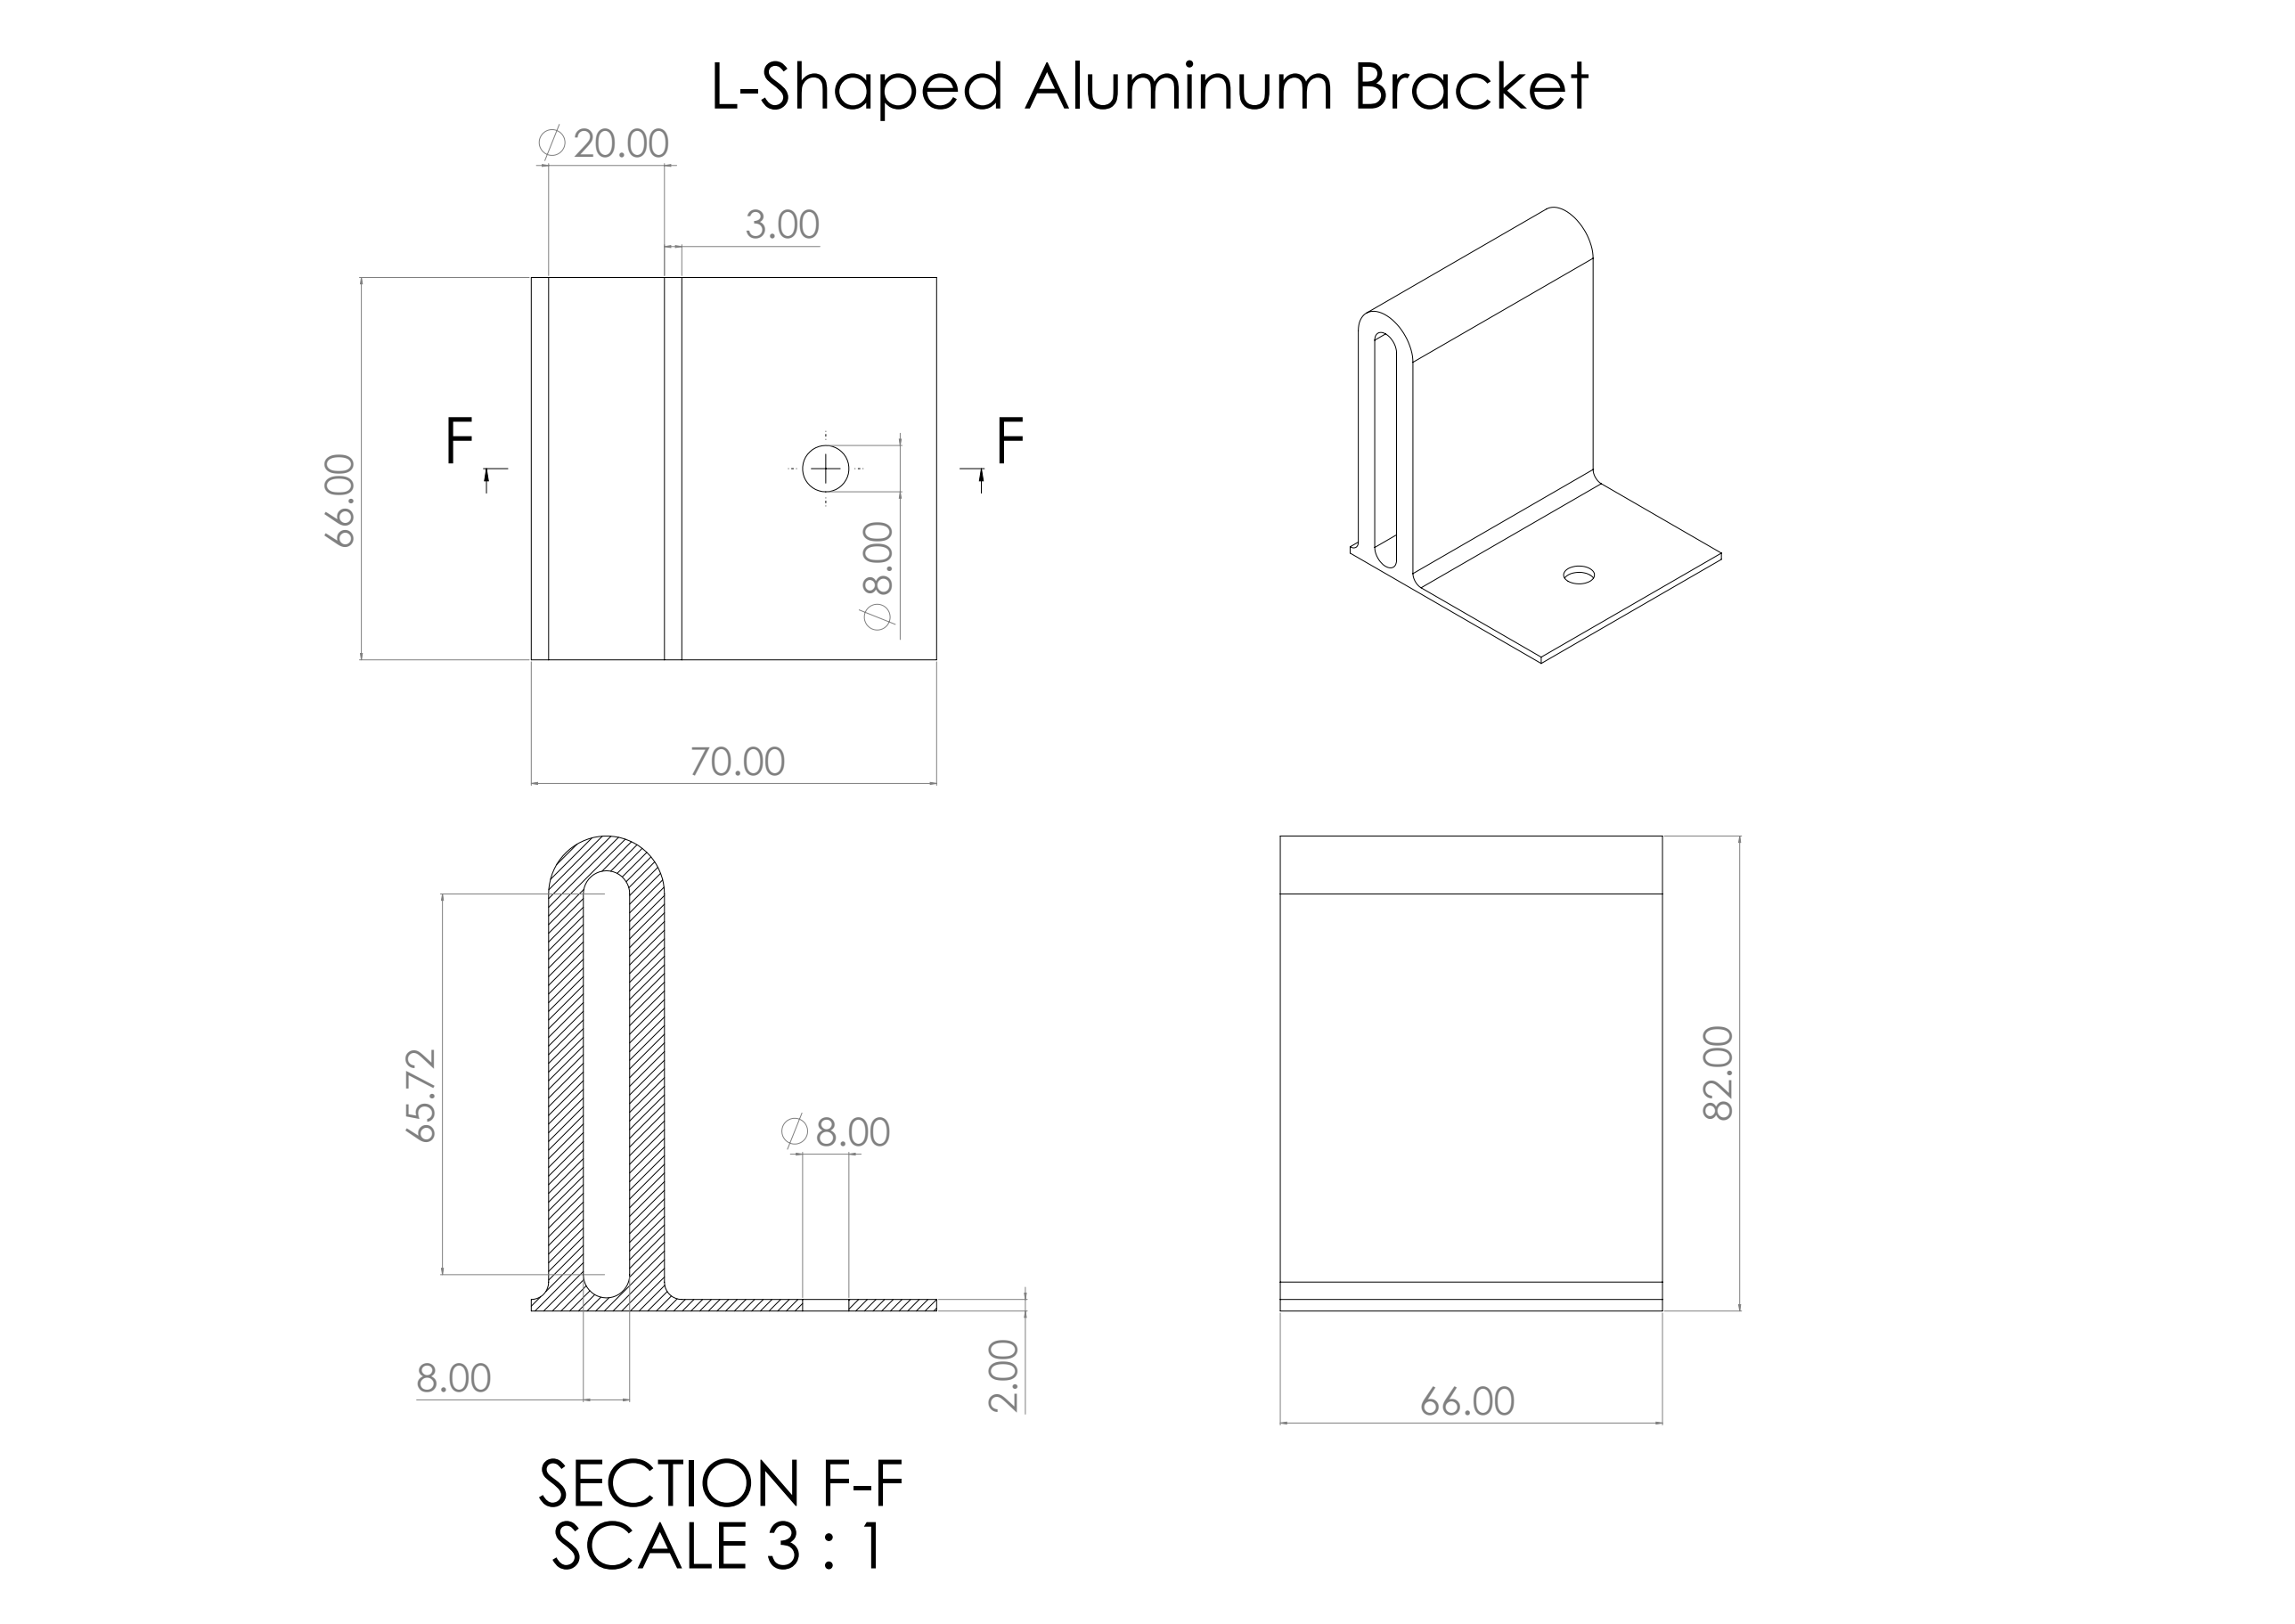
ISO-10303-21;
HEADER;
FILE_DESCRIPTION (('STEP AP214'),
    '1' );
FILE_NAME ('L-Shaped Aluminum Bracket.step',
    '2026-10-24T21:31:31',
    ( '' ),
    ( '' ),
    'SwSTEP 2.0',
    'SolidWorks 2025',
    '' );
FILE_SCHEMA (( 'AUTOMOTIVE_DESIGN' ));
ENDSEC;

DATA;
#12=EDGE_CURVE ( 'NONE', #11983, #7767, #13962, .T. ) ;
#46=PLANE ( 'NONE',  #3626 ) ;
#58=VECTOR ( 'NONE', #2580, 1000.000000000000000 ) ;
#63=DIRECTION ( 'NONE',  ( 0.000000000000000000, 1.734723475976817547E-15, -1.000000000000000000 ) ) ;
#73=EDGE_CURVE ( 'NONE', #927, #9462, #501, .T. ) ;
#97=AXIS2_PLACEMENT_3D ( 'NONE', #6521, #12302, #1688 ) ;
#99=CARTESIAN_POINT ( 'NONE',  ( 40.00000000000001421, -72.24929059928631148, -32.99999999999982947 ) ) ;
#111=FACE_OUTER_BOUND ( 'NONE', #10692, .T. ) ;
#122=EDGE_CURVE ( 'NONE', #12222, #13012, #6096, .T. ) ;
#154=DIRECTION ( 'NONE',  ( -0.000000000000000000, 1.000000000000000000, -0.000000000000000000 ) ) ;
#166=VERTEX_POINT ( 'NONE', #3346 ) ;
#182=FACE_OUTER_BOUND ( 'NONE', #8671, .T. ) ;
#200=CLOSED_SHELL ( 'NONE', ( #3830, #2727, #245, #8105, #11848, #11362, #3505, #1082, #828, #2082, #3069, #6755, #8169, #6132, #6771, #8839, #9223 ) ) ;
#204=ORIENTED_EDGE ( 'NONE', *, *, #247, .F. ) ;
#208=DIRECTION ( 'NONE',  ( -2.102695122396130409E-16, 0.000000000000000000, -1.000000000000000000 ) ) ;
#223=DIRECTION ( 'NONE',  ( 9.912705577010325549E-17, -1.734723475976817547E-15, 1.000000000000000000 ) ) ;
#245=ADVANCED_FACE ( 'NONE', ( #4003, #4739 ), #46, .F. ) ;
#247=EDGE_CURVE ( 'NONE', #8031, #13187, #10874, .T. ) ;
#263=CARTESIAN_POINT ( 'NONE',  ( -6.999999999999985789, -2.249290599286299930, -115.4621125123531442 ) ) ;
#286=VECTOR ( 'NONE', #5569, 1000.000000000000000 ) ;
#337=CARTESIAN_POINT ( 'NONE',  ( -26.99999999999998224, -72.24929059928645358, -33.00000000000000000 ) ) ;
#354=CARTESIAN_POINT ( 'NONE',  ( -29.99999999999998579, -72.24929059928631148, 33.00000000000000000 ) ) ;
#366=DIRECTION ( 'NONE',  ( 0.000000000000000000, 1.000000000000000000, 2.081668171172168119E-15 ) ) ;
#400=CARTESIAN_POINT ( 'NONE',  ( 80.00000000000001421, -72.24929059928631148, -32.99999999999999289 ) ) ;
#433=AXIS2_PLACEMENT_3D ( 'NONE', #3532, #9698, #7289 ) ;
#441=ORIENTED_EDGE ( 'NONE', *, *, #2442, .F. ) ;
#467=DIRECTION ( 'NONE',  ( 0.000000000000000000, 1.000000000000000000, 1.734723475976817547E-15 ) ) ;
#501=LINE ( 'NONE', #5201, #10269 ) ;
#520=VECTOR ( 'NONE', #3953, 1000.000000000000000 ) ;
#527=ORIENTED_EDGE ( 'NONE', *, *, #4321, .T. ) ;
#533=STYLED_ITEM('',(#15244),#4356);
#555=CARTESIAN_POINT ( 'NONE',  ( 20.86173033120691045, -74.24929059928636832, -3.999999999999999112 ) ) ;
#559=( NAMED_UNIT ( * ) SI_UNIT ( $, .STERADIAN. ) SOLID_ANGLE_UNIT ( ) );
#561=EDGE_CURVE ( 'NONE', #3921, #10500, #8809, .T. ) ;
#596=DIRECTION ( 'NONE',  ( -9.912705577010325549E-17, 1.734723475976817547E-15, -1.000000000000000000 ) ) ;
#602=LINE ( 'NONE', #8916, #9558 ) ;
#709=PLANE ( 'NONE',  #9602 ) ;
#714=DIRECTION ( 'NONE',  ( 0.000000000000000000, 0.000000000000000000, 1.000000000000000000 ) ) ;
#774=CARTESIAN_POINT ( 'NONE',  ( -29.99999999999998579, -74.24929059928642516, 32.99999999999999289 ) ) ;
#780=EDGE_CURVE ( 'NONE', #1026, #927, #5885, .T. ) ;
#802=FACE_BOUND ( 'NONE', #1169, .T. ) ;
#817=ORIENTED_EDGE ( 'NONE', *, *, #5665, .F. ) ;
#828=ADVANCED_FACE ( 'NONE', ( #11712 ), #13872, .T. ) ;
#927=VERTEX_POINT ( 'NONE', #5454 ) ;
#958=DIRECTION ( 'NONE',  ( -9.912705577010325549E-17, 1.734723475976817547E-15, -1.000000000000000000 ) ) ;
#965=VERTEX_POINT ( 'NONE', #11361 ) ;
#1000=EDGE_LOOP ( 'NONE', ( #9467, #6469, #14232, #3569 ) ) ;
#1019=VECTOR ( 'NONE', #8713, 1000.000000000000000 ) ;
#1026=VERTEX_POINT ( 'NONE', #8983 ) ;
#1027=VECTOR ( 'NONE', #1162, 1000.000000000000000 ) ;
#1061=CARTESIAN_POINT ( 'NONE',  ( 20.86173033120691045, -72.24929059928631148, -3.999999999999999112 ) ) ;
#1082=ADVANCED_FACE ( 'NONE', ( #8143 ), #6990, .T. ) ;
#1084=EDGE_CURVE ( 'NONE', #4458, #166, #5687, .T. ) ;
#1100=ORIENTED_EDGE ( 'NONE', *, *, #561, .F. ) ;
#1141=DIRECTION ( 'NONE',  ( -0.000000000000000000, -1.000000000000000000, -1.734723475976817547E-15 ) ) ;
#1161=ORIENTED_EDGE ( 'NONE', *, *, #780, .F. ) ;
#1162=DIRECTION ( 'NONE',  ( 1.051347561198064835E-16, 0.000000000000000000, 1.000000000000000000 ) ) ;
#1169=EDGE_LOOP ( 'NONE', ( #1100, #441 ) ) ;
#1181=CARTESIAN_POINT ( 'NONE',  ( 20.86173033120691045, -87.24929059928631148, 0.000000000000000000 ) ) ;
#1202=DIRECTION ( 'NONE',  ( 1.000000000000000000, 3.647594591642515023E-31, -2.102695122396130409E-16 ) ) ;
#1210=ORIENTED_EDGE ( 'NONE', *, *, #3031, .T. ) ;
#1211=CARTESIAN_POINT ( 'NONE',  ( -6.999999999999987566, -2.249290599286300818, -115.4621125123531442 ) ) ;
#1212=CARTESIAN_POINT ( 'NONE',  ( -16.99999999999998579, -67.96969602390581144, -115.4621125123531442 ) ) ;
#1224=CARTESIAN_POINT ( 'NONE',  ( -30.00000000000000000, 23.95881716715930665, -32.99999999999982236 ) ) ;
#1302=ORIENTED_EDGE ( 'NONE', *, *, #11228, .F. ) ;
#1315=ORIENTED_EDGE ( 'NONE', *, *, #6502, .T. ) ;
#1345=CARTESIAN_POINT ( 'NONE',  ( -12.99999999999998757, -2.249290599286444703, -32.99999999999987921 ) ) ;
#1422=AXIS2_PLACEMENT_3D ( 'NONE', #9838, #14588, #4037 ) ;
#1431=LINE ( 'NONE', #1654, #13791 ) ;
#1493=( LENGTH_UNIT ( ) NAMED_UNIT ( * ) SI_UNIT ( .MILLI., .METRE. ) );
#1522=CIRCLE ( 'NONE', #14296, 10.00000000000000178 ) ;
#1576=CARTESIAN_POINT ( 'NONE',  ( -6.999999999999978684, -69.24929059928631148, -32.99999999999999289 ) ) ;
#1624=CARTESIAN_POINT ( 'NONE',  ( -20.99999999999998579, -2.249290599286445591, -32.99999999999987921 ) ) ;
#1654=CARTESIAN_POINT ( 'NONE',  ( 40.00000000000002132, 23.95881716715919652, 33.00000000000017053 ) ) ;
#1658=ORIENTED_EDGE ( 'NONE', *, *, #11767, .F. ) ;
#1688=DIRECTION ( 'NONE',  ( 0.000000000000000000, 1.000000000000000000, 1.734723475976807094E-15 ) ) ;
#1716=DIRECTION ( 'NONE',  ( 0.000000000000000000, -1.000000000000000000, -2.312964634635740689E-15 ) ) ;
#1725=CIRCLE ( 'NONE', #14018, 3.000000000000002665 ) ;
#1728=ORIENTED_EDGE ( 'NONE', *, *, #247, .T. ) ;
#1747=CARTESIAN_POINT ( 'NONE',  ( 40.00000000000001421, 23.95881716715930665, -32.99999999999982947 ) ) ;
#1821=DIRECTION ( 'NONE',  ( 0.000000000000000000, 0.000000000000000000, 1.000000000000000000 ) ) ;
#1870=DIRECTION ( 'NONE',  ( -1.051347561198064835E-16, 1.682156097916903736E-15, -1.000000000000000000 ) ) ;
#2046=ORIENTED_EDGE ( 'NONE', *, *, #8831, .F. ) ;
#2067=ORIENTED_EDGE ( 'NONE', *, *, #10207, .F. ) ;
#2082=ADVANCED_FACE ( 'NONE', ( #14130 ), #2348, .T. ) ;
#2098=VECTOR ( 'NONE', #13951, 1000.000000000000000 ) ;
#2168=DIRECTION ( 'NONE',  ( 0.000000000000000000, 0.000000000000000000, 1.000000000000000000 ) ) ;
#2172=CARTESIAN_POINT ( 'NONE',  ( 20.86173033120691045, -72.24929059928631148, 0.000000000000000000 ) ) ;
#2185=ORIENTED_EDGE ( 'NONE', *, *, #780, .T. ) ;
#2190=LINE ( 'NONE', #13651, #9161 ) ;
#2193=AXIS2_PLACEMENT_3D ( 'NONE', #9260, #3255, #9025 ) ;
#2234=CARTESIAN_POINT ( 'NONE',  ( -20.99999999999998579, -67.96969602390581144, -32.99999999999998579 ) ) ;
#2255=CARTESIAN_POINT ( 'NONE',  ( 20.86173033120691045, -74.24929059928636832, 3.999999999999999112 ) ) ;
#2280=VERTEX_POINT ( 'NONE', #2234 ) ;
#2303=EDGE_LOOP ( 'NONE', ( #5933, #14533, #2769, #11027 ) ) ;
#2348=PLANE ( 'NONE',  #6120 ) ;
#2403=CARTESIAN_POINT ( 'NONE',  ( -6.999999999999978684, -69.24929059928631148, 33.00000000000000711 ) ) ;
#2420=ORIENTED_EDGE ( 'NONE', *, *, #3031, .F. ) ;
#2442=EDGE_CURVE ( 'NONE', #10500, #3921, #13064, .T. ) ;
#2445=CARTESIAN_POINT ( 'NONE',  ( -20.99999999999998579, -67.96969602390581144, -115.4621125123531442 ) ) ;
#2451=ORIENTED_EDGE ( 'NONE', *, *, #6579, .T. ) ;
#2475=ORIENTED_EDGE ( 'NONE', *, *, #7070, .F. ) ;
#2580=DIRECTION ( 'NONE',  ( 0.000000000000000000, -1.000000000000000000, -1.734723475976817547E-15 ) ) ;
#2610=ORIENTED_EDGE ( 'NONE', *, *, #13697, .F. ) ;
#2654=LINE ( 'NONE', #13195, #3969 ) ;
#2657=AXIS2_PLACEMENT_3D ( 'NONE', #13816, #958, #13740 ) ;
#2693=CARTESIAN_POINT ( 'NONE',  ( 20.86173033120691045, -74.24929059928636832, 0.000000000000000000 ) ) ;
#2727=ADVANCED_FACE ( 'NONE', ( #802, #13895 ), #5587, .T. ) ;
#2742=AXIS2_PLACEMENT_3D ( 'NONE', #12942, #12000, #10937 ) ;
#2744=DIRECTION ( 'NONE',  ( 0.000000000000000000, 1.734723475976817547E-15, -1.000000000000000000 ) ) ;
#2763=DIRECTION ( 'NONE',  ( 1.051347561198064835E-16, 0.000000000000000000, 1.000000000000000000 ) ) ;
#2769=ORIENTED_EDGE ( 'NONE', *, *, #10207, .T. ) ;
#2863=( LENGTH_UNIT ( ) NAMED_UNIT ( * ) SI_UNIT ( .MILLI., .METRE. ) );
#2902=DIRECTION ( 'NONE',  ( 0.000000000000000000, 1.734723475976817547E-15, -1.000000000000000000 ) ) ;
#2958=EDGE_LOOP ( 'NONE', ( #7879, #14398, #10143, #14155, #8547, #1210, #8196, #2978, #2185 ) ) ;
#2978=ORIENTED_EDGE ( 'NONE', *, *, #11176, .T. ) ;
#2982=CYLINDRICAL_SURFACE ( 'NONE', #15001, 2.999999999999999112 ) ;
#2999=CARTESIAN_POINT ( 'NONE',  ( -6.999999999999987566, -2.249290599286157821, 33.00000000000012790 ) ) ;
#3027=VERTEX_POINT ( 'NONE', #1576 ) ;
#3031=EDGE_CURVE ( 'NONE', #3027, #4458, #13994, .T. ) ;
#3040=VERTEX_POINT ( 'NONE', #12340 ) ;
#3047=DIRECTION ( 'NONE',  ( 2.102695122396130163E-16, -1.682156097916904130E-15, 1.000000000000000000 ) ) ;
#3069=ADVANCED_FACE ( 'NONE', ( #9190 ), #15111, .F. ) ;
#3142=ORIENTED_EDGE ( 'NONE', *, *, #13697, .T. ) ;
#3198=ORIENTED_EDGE ( 'NONE', *, *, #14960, .T. ) ;
#3227=AXIS2_PLACEMENT_3D ( 'NONE', #4760, #9745, #4598 ) ;
#3255=DIRECTION ( 'NONE',  ( -1.000000000000000000, 0.000000000000000000, 0.000000000000000000 ) ) ;
#3261=PRODUCT_DEFINITION ( 'UNKNOWN', '', #14928, #10440 ) ;
#3291=ORIENTED_EDGE ( 'NONE', *, *, #73, .T. ) ;
#3327=DIRECTION ( 'NONE',  ( 0.000000000000000000, 0.000000000000000000, 1.000000000000000000 ) ) ;
#3346=CARTESIAN_POINT ( 'NONE',  ( 40.00000000000001421, -72.24929059928631148, -32.99999999999999289 ) ) ;
#3408=CARTESIAN_POINT ( 'NONE',  ( -16.99999999999998579, -2.249290599286305703, -115.4621125123531442 ) ) ;
#3427=DIRECTION ( 'NONE',  ( 0.000000000000000000, -1.000000000000000000, -1.734723475976807094E-15 ) ) ;
#3484=DIRECTION ( 'NONE',  ( -1.000000000000000000, 0.000000000000000000, 9.912705577010325549E-17 ) ) ;
#3505=ADVANCED_FACE ( 'NONE', ( #9807, #182 ), #14348, .F. ) ;
#3532=CARTESIAN_POINT ( 'NONE',  ( -3.999999999999976019, -69.24929059928631148, -32.99999999999999289 ) ) ;
#3552=ORIENTED_EDGE ( 'NONE', *, *, #7518, .T. ) ;
#3564=CYLINDRICAL_SURFACE ( 'NONE', #7608, 3.999999999999999112 ) ;
#3569=ORIENTED_EDGE ( 'NONE', *, *, #14929, .T. ) ;
#3603=CARTESIAN_POINT ( 'NONE',  ( -29.99999999999998224, -69.24929059928631148, -32.99999999999998579 ) ) ;
#3626=AXIS2_PLACEMENT_3D ( 'NONE', #8701, #14129, #13391 ) ;
#3717=ORIENTED_EDGE ( 'NONE', *, *, #7737, .F. ) ;
#3801=LINE ( 'NONE', #8505, #1019 ) ;
#3830=ADVANCED_FACE ( 'NONE', ( #13277 ), #12119, .F. ) ;
#3845=VECTOR ( 'NONE', #14312, 1000.000000000000000 ) ;
#3854=EDGE_CURVE ( 'NONE', #2280, #3040, #11678, .T. ) ;
#3921=VERTEX_POINT ( 'NONE', #2255 ) ;
#3953=DIRECTION ( 'NONE',  ( -0.000000000000000000, 1.000000000000000000, -0.000000000000000000 ) ) ;
#3969=VECTOR ( 'NONE', #11032, 1000.000000000000000 ) ;
#4003=FACE_OUTER_BOUND ( 'NONE', #12412, .T. ) ;
#4018=CARTESIAN_POINT ( 'NONE',  ( -3.999999999999976019, -72.24929059928631148, -32.99999999999998579 ) ) ;
#4034=EDGE_CURVE ( 'NONE', #8031, #9462, #9263, .T. ) ;
#4037=DIRECTION ( 'NONE',  ( 0.000000000000000000, 1.000000000000000000, 2.312964634635740689E-15 ) ) ;
#4082=CARTESIAN_POINT ( 'NONE',  ( 0.000000000000000000, 0.000000000000000000, 0.000000000000000000 ) ) ;
#4102=CARTESIAN_POINT ( 'NONE',  ( -26.99999999999998224, -69.24929059928631148, 33.00000000000000711 ) ) ;
#4113=VECTOR ( 'NONE', #7000, 1000.000000000000000 ) ;
#4139=ORIENTED_EDGE ( 'NONE', *, *, #14960, .F. ) ;
#4160=CARTESIAN_POINT ( 'NONE',  ( -12.99999999999998757, -2.249290599286301706, 33.00000000000009948 ) ) ;
#4188=ORIENTED_EDGE ( 'NONE', *, *, #12428, .F. ) ;
#4195=CARTESIAN_POINT ( 'NONE',  ( -29.99999999999998224, -69.24929059928631148, 33.00000000000000000 ) ) ;
#4228=EDGE_CURVE ( 'NONE', #13012, #8978, #11889, .T. ) ;
#4232=EDGE_CURVE ( 'NONE', #9462, #5523, #2654, .T. ) ;
#4321=EDGE_CURVE ( 'NONE', #3040, #965, #3801, .T. ) ;
#4356=MANIFOLD_SOLID_BREP ( 'Cut-Extrude1', #200 ) ;
#4359=AXIS2_PLACEMENT_3D ( 'NONE', #11974, #2744, #366 ) ;
#4368=DIRECTION ( 'NONE',  ( 0.000000000000000000, 1.000000000000000000, 0.000000000000000000 ) ) ;
#4441=VECTOR ( 'NONE', #6738, 1000.000000000000000 ) ;
#4458=VERTEX_POINT ( 'NONE', #4018 ) ;
#4485=VECTOR ( 'NONE', #1141, 1000.000000000000000 ) ;
#4493=CARTESIAN_POINT ( 'NONE',  ( 40.00000000000002132, -72.24929059928631148, 33.00000000000000000 ) ) ;
#4545=DIRECTION ( 'NONE',  ( 1.000000000000000000, 0.000000000000000000, 0.000000000000000000 ) ) ;
#4594=( GEOMETRIC_REPRESENTATION_CONTEXT ( 3 ) GLOBAL_UNCERTAINTY_ASSIGNED_CONTEXT ( ( #6893 ) ) GLOBAL_UNIT_ASSIGNED_CONTEXT ( ( #1493, #13402, #10888 ) ) REPRESENTATION_CONTEXT ( 'NONE', 'WORKASPACE' ) );
#4598=DIRECTION ( 'NONE',  ( 0.000000000000000000, 0.000000000000000000, 1.000000000000000000 ) ) ;
#4605=CARTESIAN_POINT ( 'NONE',  ( -6.999999999999987566, -2.249290599286443815, -32.99999999999987921 ) ) ;
#4727=EDGE_LOOP ( 'NONE', ( #2420, #10789, #13026, #6753 ) ) ;
#4739=FACE_BOUND ( 'NONE', #10322, .T. ) ;
#4740=DIRECTION ( 'NONE',  ( -1.000000000000000000, -9.912705577010325549E-17, 0.000000000000000000 ) ) ;
#4760=CARTESIAN_POINT ( 'NONE',  ( 20.86173033120691045, -87.24929059928631148, 0.000000000000000000 ) ) ;
#4827=DIRECTION ( 'NONE',  ( 1.000000000000000000, 1.239088197126290570E-16, -0.000000000000000000 ) ) ;
#4858=EDGE_LOOP ( 'NONE', ( #2067, #9678, #9070, #1302 ) ) ;
#4878=VERTEX_POINT ( 'NONE', #2403 ) ;
#4894=CARTESIAN_POINT ( 'NONE',  ( -30.00000000000000000, 23.95881716715930665, -32.99999999999982236 ) ) ;
#5000=FACE_OUTER_BOUND ( 'NONE', #1000, .T. ) ;
#5022=LINE ( 'NONE', #1624, #7435 ) ;
#5029=LINE ( 'NONE', #337, #13342 ) ;
#5039=EDGE_CURVE ( 'NONE', #2280, #12222, #5022, .T. ) ;
#5044=LINE ( 'NONE', #5986, #7058 ) ;
#5090=SHAPE_DEFINITION_REPRESENTATION ( #12617, #10411 ) ;
#5101=DIRECTION ( 'NONE',  ( 0.000000000000000000, -0.000000000000000000, -1.000000000000000000 ) ) ;
#5120=EDGE_LOOP ( 'NONE', ( #5219, #14772 ) ) ;
#5128=CARTESIAN_POINT ( 'NONE',  ( -26.99999999999998224, -69.24929059928631148, -32.99999999999999289 ) ) ;
#5141=VERTEX_POINT ( 'NONE', #11376 ) ;
#5144=ORIENTED_EDGE ( 'NONE', *, *, #5665, .T. ) ;
#5199=EDGE_CURVE ( 'NONE', #13187, #927, #5863, .T. ) ;
#5201=CARTESIAN_POINT ( 'NONE',  ( -30.00000000000000000, -74.24929059928631148, -32.99999999999999289 ) ) ;
#5219=ORIENTED_EDGE ( 'NONE', *, *, #11873, .F. ) ;
#5271=LINE ( 'NONE', #6279, #520 ) ;
#5449=EDGE_LOOP ( 'NONE', ( #12886, #1728, #12499, #3291 ) ) ;
#5454=CARTESIAN_POINT ( 'NONE',  ( -30.00000000000000000, -74.24929059928631148, -32.99999999999999289 ) ) ;
#5457=ORIENTED_EDGE ( 'NONE', *, *, #7541, .F. ) ;
#5458=LINE ( 'NONE', #4605, #14943 ) ;
#5519=ORIENTED_EDGE ( 'NONE', *, *, #1084, .F. ) ;
#5523=VERTEX_POINT ( 'NONE', #11276 ) ;
#5546=ORIENTED_EDGE ( 'NONE', *, *, #12, .T. ) ;
#5550=DIRECTION ( 'NONE',  ( 0.000000000000000000, 0.000000000000000000, 1.000000000000000000 ) ) ;
#5569=DIRECTION ( 'NONE',  ( -0.000000000000000000, -1.000000000000000000, -1.734723475976817547E-15 ) ) ;
#5586=AXIS2_PLACEMENT_3D ( 'NONE', #3603, #223, #9542 ) ;
#5587=PLANE ( 'NONE',  #10599 ) ;
#5597=CARTESIAN_POINT ( 'NONE',  ( -12.99999999999998757, -67.96969602390581144, -115.4621125123531442 ) ) ;
#5630=AXIS2_PLACEMENT_3D ( 'NONE', #2693, #6248, #7468 ) ;
#5631=FACE_OUTER_BOUND ( 'NONE', #2303, .T. ) ;
#5643=LINE ( 'NONE', #8185, #2098 ) ;
#5665=EDGE_CURVE ( 'NONE', #7521, #3040, #7942, .T. ) ;
#5687=LINE ( 'NONE', #9226, #14575 ) ;
#5861=EDGE_CURVE ( 'NONE', #10116, #11668, #5029, .T. ) ;
#5862=LINE ( 'NONE', #14159, #3845 ) ;
#5863=LINE ( 'NONE', #1224, #4485 ) ;
#5869=VECTOR ( 'NONE', #11366, 1000.000000000000000 ) ;
#5885=LINE ( 'NONE', #10644, #6052 ) ;
#5922=DIRECTION ( 'NONE',  ( -1.239088197126290570E-16, 1.000000000000000000, 0.000000000000000000 ) ) ;
#5923=DIRECTION ( 'NONE',  ( 1.000000000000000000, 0.000000000000000000, 0.000000000000000000 ) ) ;
#5933=ORIENTED_EDGE ( 'NONE', *, *, #7402, .F. ) ;
#5971=CARTESIAN_POINT ( 'NONE',  ( -12.99999999999998757, -2.249290599286301706, -32.99999999999987921 ) ) ;
#5986=CARTESIAN_POINT ( 'NONE',  ( -26.99999999999998224, -72.24929059928616937, 33.00000000000000000 ) ) ;
#6015=EDGE_LOOP ( 'NONE', ( #8608, #6018, #11330, #817 ) ) ;
#6016=LINE ( 'NONE', #7154, #6670 ) ;
#6018=ORIENTED_EDGE ( 'NONE', *, *, #7070, .T. ) ;
#6052=VECTOR ( 'NONE', #3484, 1000.000000000000000 ) ;
#6096=CIRCLE ( 'NONE', #12725, 4.000000000000000000 ) ;
#6120=AXIS2_PLACEMENT_3D ( 'NONE', #12905, #4740, #9595 ) ;
#6132=ADVANCED_FACE ( 'NONE', ( #5631 ), #13777, .F. ) ;
#6158=ORIENTED_EDGE ( 'NONE', *, *, #8013, .F. ) ;
#6160=ORIENTED_EDGE ( 'NONE', *, *, #12, .F. ) ;
#6208=CARTESIAN_POINT ( 'NONE',  ( -3.999999999999976019, -69.24929059928631148, -32.99999999999998579 ) ) ;
#6228=FACE_OUTER_BOUND ( 'NONE', #4727, .T. ) ;
#6248=DIRECTION ( 'NONE',  ( -0.000000000000000000, -1.000000000000000000, -1.682156097916903736E-15 ) ) ;
#6279=CARTESIAN_POINT ( 'NONE',  ( 20.86173033120691045, -87.24929059928631148, -3.999999999999999112 ) ) ;
#6315=AXIS2_PLACEMENT_3D ( 'NONE', #4082, #8567, #11096 ) ;
#6318=ORIENTED_EDGE ( 'NONE', *, *, #122, .F. ) ;
#6347=VECTOR ( 'NONE', #8688, 1000.000000000000000 ) ;
#6367=ORIENTED_EDGE ( 'NONE', *, *, #11228, .T. ) ;
#6368=DIRECTION ( 'NONE',  ( 0.000000000000000000, 1.000000000000000000, 2.312964634635740689E-15 ) ) ;
#6469=ORIENTED_EDGE ( 'NONE', *, *, #14309, .T. ) ;
#6502=EDGE_CURVE ( 'NONE', #965, #8509, #6713, .T. ) ;
#6517=CARTESIAN_POINT ( 'NONE',  ( -16.99999999999998579, -2.249290599286305703, -32.99999999999987921 ) ) ;
#6521=CARTESIAN_POINT ( 'NONE',  ( -16.99999999999998579, -2.249290599286305703, 33.00000000000012790 ) ) ;
#6540=EDGE_LOOP ( 'NONE', ( #6763, #3198, #14910, #1658 ) ) ;
#6561=FACE_OUTER_BOUND ( 'NONE', #4858, .T. ) ;
#6568=LINE ( 'NONE', #10118, #12113 ) ;
#6579=EDGE_CURVE ( 'NONE', #6582, #6752, #7708, .T. ) ;
#6582=VERTEX_POINT ( 'NONE', #1061 ) ;
#6604=LINE ( 'NONE', #2999, #6347 ) ;
#6614=CARTESIAN_POINT ( 'NONE',  ( -20.99999999999998579, -2.249290599286302594, -32.99999999999992895 ) ) ;
#6619=ORIENTED_EDGE ( 'NONE', *, *, #4321, .F. ) ;
#6623=AXIS2_PLACEMENT_3D ( 'NONE', #400, #9659, #5101 ) ;
#6632=PLANE ( 'NONE',  #14410 ) ;
#6661=ORIENTED_EDGE ( 'NONE', *, *, #12289, .T. ) ;
#6670=VECTOR ( 'NONE', #154, 1000.000000000000000 ) ;
#6713=CIRCLE ( 'NONE', #97, 4.000000000000000000 ) ;
#6738=DIRECTION ( 'NONE',  ( 0.000000000000000000, 0.000000000000000000, 1.000000000000000000 ) ) ;
#6752=VERTEX_POINT ( 'NONE', #12058 ) ;
#6753=ORIENTED_EDGE ( 'NONE', *, *, #10683, .F. ) ;
#6755=ADVANCED_FACE ( 'NONE', ( #13070 ), #9613, .F. ) ;
#6763=ORIENTED_EDGE ( 'NONE', *, *, #5861, .F. ) ;
#6771=ADVANCED_FACE ( 'NONE', ( #6228 ), #14075, .F. ) ;
#6776=ORIENTED_EDGE ( 'NONE', *, *, #561, .T. ) ;
#6862=ORIENTED_EDGE ( 'NONE', *, *, #5039, .T. ) ;
#6893=UNCERTAINTY_MEASURE_WITH_UNIT (LENGTH_MEASURE( 1.000000000000000082E-05 ), #1493, 'distance_accuracy_value', 'NONE');
#6947=CARTESIAN_POINT ( 'NONE',  ( 40.00000000000001421, 23.95881716715930665, -32.99999999999982947 ) ) ;
#6966=EDGE_CURVE ( 'NONE', #5141, #4878, #8782, .T. ) ;
#6970=DIRECTION ( 'NONE',  ( 0.000000000000000000, 1.682156097916903736E-15, -1.000000000000000000 ) ) ;
#6990=PLANE ( 'NONE',  #13584 ) ;
#7000=DIRECTION ( 'NONE',  ( -0.000000000000000000, -1.000000000000000000, -1.734723475976817547E-15 ) ) ;
#7058=VECTOR ( 'NONE', #11894, 1000.000000000000000 ) ;
#7070=EDGE_CURVE ( 'NONE', #8978, #2280, #7324, .T. ) ;
#7096=LINE ( 'NONE', #99, #1027 ) ;
#7154=CARTESIAN_POINT ( 'NONE',  ( 20.86173033120691045, -87.24929059928631148, 3.999999999999999112 ) ) ;
#7238=LINE ( 'NONE', #9999, #5869 ) ;
#7289=DIRECTION ( 'NONE',  ( 1.000000000000000000, 0.000000000000000000, 0.000000000000000000 ) ) ;
#7324=CIRCLE ( 'NONE', #2657, 4.000000000000003553 ) ;
#7352=PLANE ( 'NONE',  #14264 ) ;
#7384=EDGE_CURVE ( 'NONE', #4878, #3027, #7238, .T. ) ;
#7402=EDGE_CURVE ( 'NONE', #12222, #965, #602, .T. ) ;
#7435=VECTOR ( 'NONE', #467, 1000.000000000000000 ) ;
#7450=AXIS2_PLACEMENT_3D ( 'NONE', #9373, #63, #10372 ) ;
#7468=DIRECTION ( 'NONE',  ( 0.000000000000000000, 0.000000000000000000, -1.000000000000000000 ) ) ;
#7518=EDGE_CURVE ( 'NONE', #7767, #4878, #6604, .T. ) ;
#7521=VERTEX_POINT ( 'NONE', #11291 ) ;
#7541=EDGE_CURVE ( 'NONE', #10777, #3027, #5458, .T. ) ;
#7581=EDGE_LOOP ( 'NONE', ( #3717, #204, #2046, #4139 ) ) ;
#7608=AXIS2_PLACEMENT_3D ( 'NONE', #1181, #12893, #11554 ) ;
#7708=CIRCLE ( 'NONE', #13602, 3.999999999999999112 ) ;
#7737=EDGE_CURVE ( 'NONE', #13187, #10116, #14431, .T. ) ;
#7767=VERTEX_POINT ( 'NONE', #10688 ) ;
#7863=VERTEX_POINT ( 'NONE', #13367 ) ;
#7879=ORIENTED_EDGE ( 'NONE', *, *, #5199, .F. ) ;
#7942=CIRCLE ( 'NONE', #7450, 4.000000000000003553 ) ;
#7992=ORIENTED_EDGE ( 'NONE', *, *, #11873, .T. ) ;
#8013=EDGE_CURVE ( 'NONE', #12681, #11983, #5044, .T. ) ;
#8031=VERTEX_POINT ( 'NONE', #354 ) ;
#8105=ADVANCED_FACE ( 'NONE', ( #11813 ), #7352, .F. ) ;
#8143=FACE_OUTER_BOUND ( 'NONE', #13211, .T. ) ;
#8169=ADVANCED_FACE ( 'NONE', ( #6561 ), #709, .F. ) ;
#8185=CARTESIAN_POINT ( 'NONE',  ( -26.99999999999998934, -2.249290599286302150, -115.4621125123531442 ) ) ;
#8196=ORIENTED_EDGE ( 'NONE', *, *, #1084, .T. ) ;
#8281=AXIS2_PLACEMENT_3D ( 'NONE', #1747, #14389, #2763 ) ;
#8308=DIRECTION ( 'NONE',  ( 0.000000000000000000, 0.000000000000000000, 1.000000000000000000 ) ) ;
#8350=ORIENTED_EDGE ( 'NONE', *, *, #14929, .F. ) ;
#8455=EDGE_CURVE ( 'NONE', #10777, #7767, #10804, .T. ) ;
#8500=DIRECTION ( 'NONE',  ( 0.000000000000000000, 0.000000000000000000, 1.000000000000000000 ) ) ;
#8505=CARTESIAN_POINT ( 'NONE',  ( -20.99999999999998579, -2.249290599286159598, 33.00000000000012790 ) ) ;
#8509=VERTEX_POINT ( 'NONE', #4160 ) ;
#8547=ORIENTED_EDGE ( 'NONE', *, *, #7541, .T. ) ;
#8567=DIRECTION ( 'NONE',  ( 0.000000000000000000, 0.000000000000000000, 1.000000000000000000 ) ) ;
#8581=DIRECTION ( 'NONE',  ( -0.000000000000000000, -1.000000000000000000, -1.734723475976817547E-15 ) ) ;
#8602=ORIENTED_EDGE ( 'NONE', *, *, #13924, .F. ) ;
#8608=ORIENTED_EDGE ( 'NONE', *, *, #13520, .F. ) ;
#8671=EDGE_LOOP ( 'NONE', ( #5519, #10673, #8602, #11585 ) ) ;
#8674=FACE_OUTER_BOUND ( 'NONE', #7581, .T. ) ;
#8688=DIRECTION ( 'NONE',  ( 1.239088197126290570E-16, -1.000000000000000000, -1.734723475976817744E-15 ) ) ;
#8701=CARTESIAN_POINT ( 'NONE',  ( 40.00000000000002132, 23.95881716715919652, 33.00000000000017053 ) ) ;
#8713=DIRECTION ( 'NONE',  ( 0.000000000000000000, 1.000000000000000000, 1.734723475976817744E-15 ) ) ;
#8737=ORIENTED_EDGE ( 'NONE', *, *, #12289, .F. ) ;
#8782=CIRCLE ( 'NONE', #1422, 3.000000000000002665 ) ;
#8809=CIRCLE ( 'NONE', #5630, 3.999999999999999112 ) ;
#8831=EDGE_CURVE ( 'NONE', #12681, #8031, #1725, .T. ) ;
#8839=ADVANCED_FACE ( 'NONE', ( #8674 ), #2982, .F. ) ;
#8916=CARTESIAN_POINT ( 'NONE',  ( -20.99999999999998579, -2.249290599286302594, -115.4621125123531442 ) ) ;
#8978=VERTEX_POINT ( 'NONE', #10186 ) ;
#8983=CARTESIAN_POINT ( 'NONE',  ( 40.00000000000001421, -74.24929059928631148, -33.00000000000000000 ) ) ;
#9025=DIRECTION ( 'NONE',  ( 0.000000000000000000, 0.000000000000000000, 1.000000000000000000 ) ) ;
#9070=ORIENTED_EDGE ( 'NONE', *, *, #13520, .T. ) ;
#9128=CARTESIAN_POINT ( 'NONE',  ( 0.000000000000000000, -74.24929059928636832, -1.248988969475937798E-13 ) ) ;
#9161=VECTOR ( 'NONE', #1870, 1000.000000000000000 ) ;
#9190=FACE_OUTER_BOUND ( 'NONE', #15147, .T. ) ;
#9204=CARTESIAN_POINT ( 'NONE',  ( -12.99999999999998757, -2.249290599286301706, -115.4621125123531442 ) ) ;
#9223=ADVANCED_FACE ( 'NONE', ( #111 ), #3564, .F. ) ;
#9226=CARTESIAN_POINT ( 'NONE',  ( 40.00000000000001421, -72.24929059928631148, -32.99999999999999289 ) ) ;
#9260=CARTESIAN_POINT ( 'NONE',  ( -20.99999999999998579, -2.249290599286302594, -115.4621125123531442 ) ) ;
#9263=LINE ( 'NONE', #11401, #286 ) ;
#9282=VECTOR ( 'NONE', #13472, 1000.000000000000000 ) ;
#9305=DIRECTION ( 'NONE',  ( 1.239088197126290570E-16, -1.000000000000000000, -1.734723475976817547E-15 ) ) ;
#9373=CARTESIAN_POINT ( 'NONE',  ( -16.99999999999998579, -67.96969602390581144, 33.00000000000001421 ) ) ;
#9424=EDGE_LOOP ( 'NONE', ( #12721, #2475, #11408, #6318 ) ) ;
#9462=VERTEX_POINT ( 'NONE', #774 ) ;
#9467=ORIENTED_EDGE ( 'NONE', *, *, #11176, .F. ) ;
#9533=APPLICATION_CONTEXT ( 'automotive_design' ) ;
#9542=DIRECTION ( 'NONE',  ( 0.000000000000000000, -1.000000000000000000, -2.312964634635740689E-15 ) ) ;
#9551=VECTOR ( 'NONE', #2168, 1000.000000000000000 ) ;
#9558=VECTOR ( 'NONE', #12383, 1000.000000000000000 ) ;
#9595=DIRECTION ( 'NONE',  ( 9.912705577010325549E-17, -1.000000000000000000, 0.000000000000000000 ) ) ;
#9602=AXIS2_PLACEMENT_3D ( 'NONE', #12344, #11254, #13348 ) ;
#9613=CYLINDRICAL_SURFACE ( 'NONE', #12980, 4.000000000000000000 ) ;
#9659=DIRECTION ( 'NONE',  ( 0.000000000000000000, -1.000000000000000000, 0.000000000000000000 ) ) ;
#9678=ORIENTED_EDGE ( 'NONE', *, *, #4228, .T. ) ;
#9681=UNCERTAINTY_MEASURE_WITH_UNIT (LENGTH_MEASURE( 1.000000000000000082E-05 ), #2863, 'distance_accuracy_value', 'NONE');
#9698=DIRECTION ( 'NONE',  ( 0.000000000000000000, 0.000000000000000000, 1.000000000000000000 ) ) ;
#9706=PLANE ( 'NONE',  #8281 ) ;
#9745=DIRECTION ( 'NONE',  ( -0.000000000000000000, 1.000000000000000000, -0.000000000000000000 ) ) ;
#9746=AXIS2_PLACEMENT_3D ( 'NONE', #2172, #11549, #15029 ) ;
#9807=FACE_BOUND ( 'NONE', #5120, .T. ) ;
#9816=CARTESIAN_POINT ( 'NONE',  ( -26.99999999999998934, -2.249290599286302150, -32.99999999999987921 ) ) ;
#9838=CARTESIAN_POINT ( 'NONE',  ( -3.999999999999976019, -69.24929059928631148, 33.00000000000000711 ) ) ;
#9862=ORIENTED_EDGE ( 'NONE', *, *, #13784, .F. ) ;
#9900=ORIENTED_EDGE ( 'NONE', *, *, #4034, .T. ) ;
#9999=CARTESIAN_POINT ( 'NONE',  ( -6.999999999999978684, -69.24929059928631148, -115.4621125123531442 ) ) ;
#10055=ORIENTED_EDGE ( 'NONE', *, *, #8455, .F. ) ;
#10116=VERTEX_POINT ( 'NONE', #5128 ) ;
#10118=CARTESIAN_POINT ( 'NONE',  ( -26.99999999999998224, -69.24929059928631148, -115.4621125123531442 ) ) ;
#10132=ORIENTED_EDGE ( 'NONE', *, *, #4232, .F. ) ;
#10143=ORIENTED_EDGE ( 'NONE', *, *, #5861, .T. ) ;
#10186=CARTESIAN_POINT ( 'NONE',  ( -12.99999999999998757, -67.96969602390581144, -32.99999999999998579 ) ) ;
#10207=EDGE_CURVE ( 'NONE', #13012, #8509, #11410, .T. ) ;
#10269=VECTOR ( 'NONE', #3047, 1000.000000000000000 ) ;
#10270=ORIENTED_EDGE ( 'NONE', *, *, #7384, .T. ) ;
#10322=EDGE_LOOP ( 'NONE', ( #1315, #6367, #5144, #527 ) ) ;
#10334=FACE_OUTER_BOUND ( 'NONE', #2958, .T. ) ;
#10372=DIRECTION ( 'NONE',  ( 0.000000000000000000, 1.000000000000000000, 1.734723475976805517E-15 ) ) ;
#10411=SHAPE_REPRESENTATION ( 'L-Shaped Aluminum Bracket', ( #6315 ), #4594 ) ;
#10440=PRODUCT_DEFINITION_CONTEXT ( 'detailed design', #14881, 'design' ) ;
#10474=CARTESIAN_POINT ( 'NONE',  ( -16.99999999999998579, -2.249290599286305703, -115.4621125123531442 ) ) ;
#10500=VERTEX_POINT ( 'NONE', #555 ) ;
#10535=CARTESIAN_POINT ( 'NONE',  ( 20.86173033120691045, -72.24929059928631148, 0.000000000000000000 ) ) ;
#10599=AXIS2_PLACEMENT_3D ( 'NONE', #9128, #13812, #6970 ) ;
#10608=VECTOR ( 'NONE', #13990, 1000.000000000000000 ) ;
#10644=CARTESIAN_POINT ( 'NONE',  ( 40.00000000000001421, -74.24929059928631148, -33.00000000000000000 ) ) ;
#10673=ORIENTED_EDGE ( 'NONE', *, *, #10683, .T. ) ;
#10683=EDGE_CURVE ( 'NONE', #4458, #5141, #14862, .T. ) ;
#10688=CARTESIAN_POINT ( 'NONE',  ( -6.999999999999985789, -2.249290599286299930, 33.00000000000012790 ) ) ;
#10692=EDGE_LOOP ( 'NONE', ( #2610, #11988, #6661, #7992 ) ) ;
#10716=CIRCLE ( 'NONE', #9746, 3.999999999999999112 ) ;
#10771=CARTESIAN_POINT ( 'NONE',  ( 40.00000000000001421, 23.95881716715930665, -32.99999999999982947 ) ) ;
#10777=VERTEX_POINT ( 'NONE', #14945 ) ;
#10789=ORIENTED_EDGE ( 'NONE', *, *, #7384, .F. ) ;
#10804=LINE ( 'NONE', #263, #11539 ) ;
#10874=LINE ( 'NONE', #14412, #9282 ) ;
#10888=( NAMED_UNIT ( * ) SI_UNIT ( $, .STERADIAN. ) SOLID_ANGLE_UNIT ( ) );
#10937=DIRECTION ( 'NONE',  ( 0.000000000000000000, 0.000000000000000000, -1.000000000000000000 ) ) ;
#11027=ORIENTED_EDGE ( 'NONE', *, *, #6502, .F. ) ;
#11032=DIRECTION ( 'NONE',  ( 1.000000000000000000, -0.000000000000000000, -0.000000000000000000 ) ) ;
#11087=ORIENTED_EDGE ( 'NONE', *, *, #7402, .T. ) ;
#11096=DIRECTION ( 'NONE',  ( 1.000000000000000000, 0.000000000000000000, 0.000000000000000000 ) ) ;
#11143=DIRECTION ( 'NONE',  ( 0.000000000000000000, -1.000000000000000000, -2.081668171172168119E-15 ) ) ;
#11176=EDGE_CURVE ( 'NONE', #166, #1026, #15156, .T. ) ;
#11228=EDGE_CURVE ( 'NONE', #8509, #7521, #5862, .T. ) ;
#11254=DIRECTION ( 'NONE',  ( 1.000000000000000000, 0.000000000000000000, -0.000000000000000000 ) ) ;
#11269=ORIENTED_EDGE ( 'NONE', *, *, #7518, .F. ) ;
#11276=CARTESIAN_POINT ( 'NONE',  ( 40.00000000000002132, -74.24929059928642516, 32.99999999999999289 ) ) ;
#11291=CARTESIAN_POINT ( 'NONE',  ( -12.99999999999998757, -67.96969602390581144, 33.00000000000001421 ) ) ;
#11330=ORIENTED_EDGE ( 'NONE', *, *, #3854, .T. ) ;
#11332=VECTOR ( 'NONE', #14724, 1000.000000000000000 ) ;
#11361=CARTESIAN_POINT ( 'NONE',  ( -20.99999999999998579, -2.249290599286302594, 33.00000000000012790 ) ) ;
#11362=ADVANCED_FACE ( 'NONE', ( #5000 ), #9706, .F. ) ;
#11366=DIRECTION ( 'NONE',  ( -0.000000000000000000, -0.000000000000000000, -1.000000000000000000 ) ) ;
#11376=CARTESIAN_POINT ( 'NONE',  ( -3.999999999999976019, -72.24929059928631148, 33.00000000000000000 ) ) ;
#11401=CARTESIAN_POINT ( 'NONE',  ( -29.99999999999998579, 23.95881716715919652, 33.00000000000017053 ) ) ;
#11408=ORIENTED_EDGE ( 'NONE', *, *, #4228, .F. ) ;
#11410=LINE ( 'NONE', #9204, #15160 ) ;
#11491=DIRECTION ( 'NONE',  ( 0.000000000000000000, 0.000000000000000000, 1.000000000000000000 ) ) ;
#11518=DIRECTION ( 'NONE',  ( 0.000000000000000000, 0.000000000000000000, 1.000000000000000000 ) ) ;
#11519=AXIS2_PLACEMENT_3D ( 'NONE', #6208, #12261, #1716 ) ;
#11539=VECTOR ( 'NONE', #8500, 1000.000000000000000 ) ;
#11549=DIRECTION ( 'NONE',  ( 0.000000000000000000, 1.000000000000000000, 0.000000000000000000 ) ) ;
#11550=DIRECTION ( 'NONE',  ( 1.000000000000000000, 0.000000000000000000, 0.000000000000000000 ) ) ;
#11554=DIRECTION ( 'NONE',  ( 0.000000000000000000, 0.000000000000000000, 1.000000000000000000 ) ) ;
#11575=CARTESIAN_POINT ( 'NONE',  ( -16.99999999999998579, -2.249290599286305703, -32.99999999999987921 ) ) ;
#11585=ORIENTED_EDGE ( 'NONE', *, *, #14309, .F. ) ;
#11668=VERTEX_POINT ( 'NONE', #9816 ) ;
#11678=LINE ( 'NONE', #2445, #10608 ) ;
#11680=DIRECTION ( 'NONE',  ( 1.000000000000000000, 0.000000000000000000, -9.912705577010325549E-17 ) ) ;
#11712=FACE_OUTER_BOUND ( 'NONE', #13370, .T. ) ;
#11767=EDGE_CURVE ( 'NONE', #11668, #11983, #5643, .T. ) ;
#11813=FACE_OUTER_BOUND ( 'NONE', #5449, .T. ) ;
#11848=ADVANCED_FACE ( 'NONE', ( #10334, #13719 ), #6632, .F. ) ;
#11873=EDGE_CURVE ( 'NONE', #6752, #6582, #10716, .T. ) ;
#11889=LINE ( 'NONE', #1345, #58 ) ;
#11894=DIRECTION ( 'NONE',  ( -9.912705577010326782E-17, 1.000000000000000000, 1.734723475976817744E-15 ) ) ;
#11974=CARTESIAN_POINT ( 'NONE',  ( -16.99999999999998579, -2.249290599286305703, 33.00000000000012790 ) ) ;
#11983=VERTEX_POINT ( 'NONE', #14184 ) ;
#11988=ORIENTED_EDGE ( 'NONE', *, *, #2442, .T. ) ;
#12000=DIRECTION ( 'NONE',  ( -0.000000000000000000, -1.000000000000000000, -1.682156097916903736E-15 ) ) ;
#12058=CARTESIAN_POINT ( 'NONE',  ( 20.86173033120691045, -72.24929059928631148, 3.999999999999999112 ) ) ;
#12113=VECTOR ( 'NONE', #714, 1000.000000000000000 ) ;
#12119=CYLINDRICAL_SURFACE ( 'NONE', #3227, 3.999999999999999112 ) ;
#12210=ORIENTED_EDGE ( 'NONE', *, *, #8455, .T. ) ;
#12222=VERTEX_POINT ( 'NONE', #6614 ) ;
#12260=( NAMED_UNIT ( * ) PLANE_ANGLE_UNIT ( ) SI_UNIT ( $, .RADIAN. ) );
#12261=DIRECTION ( 'NONE',  ( 9.912705577010325549E-17, -1.734723475976817547E-15, 1.000000000000000000 ) ) ;
#12289=EDGE_CURVE ( 'NONE', #3921, #6752, #6016, .T. ) ;
#12302=DIRECTION ( 'NONE',  ( 0.000000000000000000, 1.734723475976817547E-15, -1.000000000000000000 ) ) ;
#12340=CARTESIAN_POINT ( 'NONE',  ( -20.99999999999998579, -67.96969602390581144, 33.00000000000001421 ) ) ;
#12344=CARTESIAN_POINT ( 'NONE',  ( -12.99999999999998757, -2.249290599286301706, -115.4621125123531442 ) ) ;
#12369=CARTESIAN_POINT ( 'NONE',  ( -29.99999999999998224, -69.24929059928631148, -115.4621125123531442 ) ) ;
#12383=DIRECTION ( 'NONE',  ( 0.000000000000000000, 0.000000000000000000, 1.000000000000000000 ) ) ;
#12412=EDGE_LOOP ( 'NONE', ( #9862, #15193, #12900, #11269, #6160, #6158, #12936, #9900, #14194 ) ) ;
#12428=EDGE_CURVE ( 'NONE', #11668, #10777, #1522, .T. ) ;
#12485=CARTESIAN_POINT ( 'NONE',  ( -3.999999999999976019, -72.24929059928631148, -32.99999999999999289 ) ) ;
#12499=ORIENTED_EDGE ( 'NONE', *, *, #5199, .T. ) ;
#12617=PRODUCT_DEFINITION_SHAPE ( 'NONE', 'NONE',  #3261 ) ;
#12681=VERTEX_POINT ( 'NONE', #4102 ) ;
#12721=ORIENTED_EDGE ( 'NONE', *, *, #5039, .F. ) ;
#12725=AXIS2_PLACEMENT_3D ( 'NONE', #11575, #12904, #3427 ) ;
#12843=AXIS2_PLACEMENT_3D ( 'NONE', #3408, #3327, #11550 ) ;
#12882=EDGE_LOOP ( 'NONE', ( #8350, #10132, #13854, #1161 ) ) ;
#12886=ORIENTED_EDGE ( 'NONE', *, *, #4034, .F. ) ;
#12893=DIRECTION ( 'NONE',  ( -0.000000000000000000, 1.000000000000000000, -0.000000000000000000 ) ) ;
#12900=ORIENTED_EDGE ( 'NONE', *, *, #6966, .T. ) ;
#12904=DIRECTION ( 'NONE',  ( -9.912705577010325549E-17, 1.734723475976817547E-15, -1.000000000000000000 ) ) ;
#12905=CARTESIAN_POINT ( 'NONE',  ( -26.99999999999998224, -72.24929059928631148, -115.4621125123531442 ) ) ;
#12936=ORIENTED_EDGE ( 'NONE', *, *, #8831, .T. ) ;
#12942=CARTESIAN_POINT ( 'NONE',  ( 20.86173033120691045, -74.24929059928636832, 0.000000000000000000 ) ) ;
#12980=AXIS2_PLACEMENT_3D ( 'NONE', #1212, #8308, #5923 ) ;
#13012=VERTEX_POINT ( 'NONE', #5971 ) ;
#13026=ORIENTED_EDGE ( 'NONE', *, *, #6966, .F. ) ;
#13064=CIRCLE ( 'NONE', #2742, 3.999999999999999112 ) ;
#13070=FACE_OUTER_BOUND ( 'NONE', #6015, .T. ) ;
#13137=ORIENTED_EDGE ( 'NONE', *, *, #3854, .F. ) ;
#13171=PRODUCT_CONTEXT ( 'NONE', #9533, 'mechanical' ) ;
#13187=VERTEX_POINT ( 'NONE', #13764 ) ;
#13195=CARTESIAN_POINT ( 'NONE',  ( 40.00000000000002132, -74.24929059928642516, 32.99999999999999289 ) ) ;
#13211=EDGE_LOOP ( 'NONE', ( #3552, #10270, #5457, #12210 ) ) ;
#13277=FACE_OUTER_BOUND ( 'NONE', #13860, .T. ) ;
#13342=VECTOR ( 'NONE', #14486, 1000.000000000000000 ) ;
#13348=DIRECTION ( 'NONE',  ( -0.000000000000000000, 0.000000000000000000, -1.000000000000000000 ) ) ;
#13367=CARTESIAN_POINT ( 'NONE',  ( 40.00000000000002132, -72.24929059928631148, 33.00000000000000000 ) ) ;
#13370=EDGE_LOOP ( 'NONE', ( #4188, #14158, #5546, #10055 ) ) ;
#13391=DIRECTION ( 'NONE',  ( 0.000000000000000000, 1.000000000000000000, 1.734723475976817547E-15 ) ) ;
#13402=( NAMED_UNIT ( * ) PLANE_ANGLE_UNIT ( ) SI_UNIT ( $, .RADIAN. ) );
#13442=ADVANCED_BREP_SHAPE_REPRESENTATION ( '', ( #4356, #6315 ), #4594 ) ;
#13472=DIRECTION ( 'NONE',  ( -2.102695122396130409E-16, 0.000000000000000000, -1.000000000000000000 ) ) ;
#13520=EDGE_CURVE ( 'NONE', #8978, #7521, #15063, .T. ) ;
#13584=AXIS2_PLACEMENT_3D ( 'NONE', #1211, #4827, #5922 ) ;
#13602=AXIS2_PLACEMENT_3D ( 'NONE', #10535, #4368, #11518 ) ;
#13651=CARTESIAN_POINT ( 'NONE',  ( 40.00000000000001421, -74.24929059928631148, -33.00000000000000000 ) ) ;
#13697=EDGE_CURVE ( 'NONE', #10500, #6582, #5271, .T. ) ;
#13719=FACE_BOUND ( 'NONE', #9424, .T. ) ;
#13740=DIRECTION ( 'NONE',  ( 0.000000000000000000, -1.000000000000000000, -1.734723475976805517E-15 ) ) ;
#13764=CARTESIAN_POINT ( 'NONE',  ( -30.00000000000000000, -72.24929059928631148, -32.99999999999999289 ) ) ;
#13777=CYLINDRICAL_SURFACE ( 'NONE', #15085, 4.000000000000000000 ) ;
#13784=EDGE_CURVE ( 'NONE', #7863, #5523, #1431, .T. ) ;
#13791=VECTOR ( 'NONE', #8581, 1000.000000000000000 ) ;
#13812=DIRECTION ( 'NONE',  ( 0.000000000000000000, -1.000000000000000000, -1.682156097916903736E-15 ) ) ;
#13816=CARTESIAN_POINT ( 'NONE',  ( -16.99999999999998579, -67.96969602390581144, -32.99999999999998579 ) ) ;
#13854=ORIENTED_EDGE ( 'NONE', *, *, #73, .F. ) ;
#13860=EDGE_LOOP ( 'NONE', ( #6776, #3142, #2451, #8737 ) ) ;
#13871=DIRECTION ( 'NONE',  ( 0.000000000000000000, -1.000000000000000000, -1.734723475976817547E-15 ) ) ;
#13872=CYLINDRICAL_SURFACE ( 'NONE', #12843, 10.00000000000000178 ) ;
#13895=FACE_OUTER_BOUND ( 'NONE', #12882, .T. ) ;
#13924=EDGE_CURVE ( 'NONE', #7863, #5141, #14800, .T. ) ;
#13951=DIRECTION ( 'NONE',  ( 0.000000000000000000, 0.000000000000000000, 1.000000000000000000 ) ) ;
#13962=CIRCLE ( 'NONE', #4359, 10.00000000000000178 ) ;
#13990=DIRECTION ( 'NONE',  ( 0.000000000000000000, 0.000000000000000000, 1.000000000000000000 ) ) ;
#13994=CIRCLE ( 'NONE', #11519, 3.000000000000002665 ) ;
#14018=AXIS2_PLACEMENT_3D ( 'NONE', #4195, #2902, #6368 ) ;
#14025=DIRECTION ( 'NONE',  ( 9.912705577010325549E-17, -1.734723475976817547E-15, 1.000000000000000000 ) ) ;
#14060=( GEOMETRIC_REPRESENTATION_CONTEXT ( 3 ) GLOBAL_UNCERTAINTY_ASSIGNED_CONTEXT ( ( #9681 ) ) GLOBAL_UNIT_ASSIGNED_CONTEXT ( ( #2863, #12260, #559 ) ) REPRESENTATION_CONTEXT ( 'NONE', 'WORKASPACE' ) );
#14075=CYLINDRICAL_SURFACE ( 'NONE', #433, 3.000000000000000000 ) ;
#14129=DIRECTION ( 'NONE',  ( 0.000000000000000000, 1.734723475976817547E-15, -1.000000000000000000 ) ) ;
#14130=FACE_OUTER_BOUND ( 'NONE', #6540, .T. ) ;
#14155=ORIENTED_EDGE ( 'NONE', *, *, #12428, .T. ) ;
#14158=ORIENTED_EDGE ( 'NONE', *, *, #11767, .T. ) ;
#14159=CARTESIAN_POINT ( 'NONE',  ( -12.99999999999998757, -2.249290599286158709, 33.00000000000012790 ) ) ;
#14184=CARTESIAN_POINT ( 'NONE',  ( -26.99999999999998934, -2.249290599286302150, 33.00000000000009948 ) ) ;
#14194=ORIENTED_EDGE ( 'NONE', *, *, #4232, .T. ) ;
#14232=ORIENTED_EDGE ( 'NONE', *, *, #13784, .T. ) ;
#14264=AXIS2_PLACEMENT_3D ( 'NONE', #4894, #1202, #208 ) ;
#14296=AXIS2_PLACEMENT_3D ( 'NONE', #6517, #596, #11143 ) ;
#14309=EDGE_CURVE ( 'NONE', #166, #7863, #7096, .T. ) ;
#14312=DIRECTION ( 'NONE',  ( 0.000000000000000000, -1.000000000000000000, -1.734723475976817744E-15 ) ) ;
#14316=MECHANICAL_DESIGN_GEOMETRIC_PRESENTATION_REPRESENTATION('',(#533),#14060);
#14348=PLANE ( 'NONE',  #6623 ) ;
#14389=DIRECTION ( 'NONE',  ( -1.000000000000000000, -1.823797295821256855E-31, 1.051347561198064835E-16 ) ) ;
#14398=ORIENTED_EDGE ( 'NONE', *, *, #7737, .T. ) ;
#14410=AXIS2_PLACEMENT_3D ( 'NONE', #6947, #14025, #13871 ) ;
#14412=CARTESIAN_POINT ( 'NONE',  ( -30.00000000000000000, -72.24929059928631148, -32.99999999999982236 ) ) ;
#14431=CIRCLE ( 'NONE', #5586, 3.000000000000002665 ) ;
#14486=DIRECTION ( 'NONE',  ( -9.912705577010325549E-17, 1.000000000000000000, 1.734723475976817547E-15 ) ) ;
#14533=ORIENTED_EDGE ( 'NONE', *, *, #122, .T. ) ;
#14566=SHAPE_REPRESENTATION_RELATIONSHIP ( 'NONE' , 'NONE' ,  #10411, #13442 ) ;
#14575=VECTOR ( 'NONE', #11680, 1000.000000000000000 ) ;
#14588=DIRECTION ( 'NONE',  ( 0.000000000000000000, 1.734723475976817547E-15, -1.000000000000000000 ) ) ;
#14724=DIRECTION ( 'NONE',  ( -1.000000000000000000, 0.000000000000000000, 0.000000000000000000 ) ) ;
#14744=DIRECTION ( 'NONE',  ( 1.000000000000000000, 0.000000000000000000, 0.000000000000000000 ) ) ;
#14772=ORIENTED_EDGE ( 'NONE', *, *, #6579, .F. ) ;
#14800=LINE ( 'NONE', #4493, #11332 ) ;
#14862=LINE ( 'NONE', #12485, #9551 ) ;
#14881=APPLICATION_CONTEXT ( 'automotive_design' ) ;
#14910=ORIENTED_EDGE ( 'NONE', *, *, #8013, .T. ) ;
#14928=PRODUCT_DEFINITION_FORMATION_WITH_SPECIFIED_SOURCE ( 'ANY', '', #14949, .NOT_KNOWN. ) ;
#14929=EDGE_CURVE ( 'NONE', #5523, #1026, #2190, .T. ) ;
#14943=VECTOR ( 'NONE', #9305, 1000.000000000000000 ) ;
#14945=CARTESIAN_POINT ( 'NONE',  ( -6.999999999999985789, -2.249290599286299930, -32.99999999999994316 ) ) ;
#14949=PRODUCT ( 'L-Shaped Aluminum Bracket', 'L-Shaped Aluminum Bracket', '', ( #13171 ) ) ;
#14960=EDGE_CURVE ( 'NONE', #10116, #12681, #6568, .T. ) ;
#15001=AXIS2_PLACEMENT_3D ( 'NONE', #12369, #1821, #14744 ) ;
#15029=DIRECTION ( 'NONE',  ( 0.000000000000000000, 0.000000000000000000, 1.000000000000000000 ) ) ;
#15063=LINE ( 'NONE', #5597, #4441 ) ;
#15085=AXIS2_PLACEMENT_3D ( 'NONE', #10474, #5550, #4545 ) ;
#15111=PLANE ( 'NONE',  #2193 ) ;
#15147=EDGE_LOOP ( 'NONE', ( #13137, #6862, #11087, #6619 ) ) ;
#15156=LINE ( 'NONE', #10771, #4113 ) ;
#15160=VECTOR ( 'NONE', #11491, 1000.000000000000000 ) ;
#15193=ORIENTED_EDGE ( 'NONE', *, *, #13924, .T. ) ;
#15238=COLOUR_RGB('Dark Blue',0.08,0.2,0.34);
#15239=FILL_AREA_STYLE_COLOUR('',#15238);
#15240=FILL_AREA_STYLE('',(#15239));
#15241=SURFACE_STYLE_FILL_AREA(#15240);
#15242=SURFACE_SIDE_STYLE('',(#15241));
#15243=SURFACE_STYLE_USAGE(.BOTH.,#15242);
#15244=PRESENTATION_STYLE_ASSIGNMENT((#15243));
ENDSEC;
END-ISO-10303-21;
